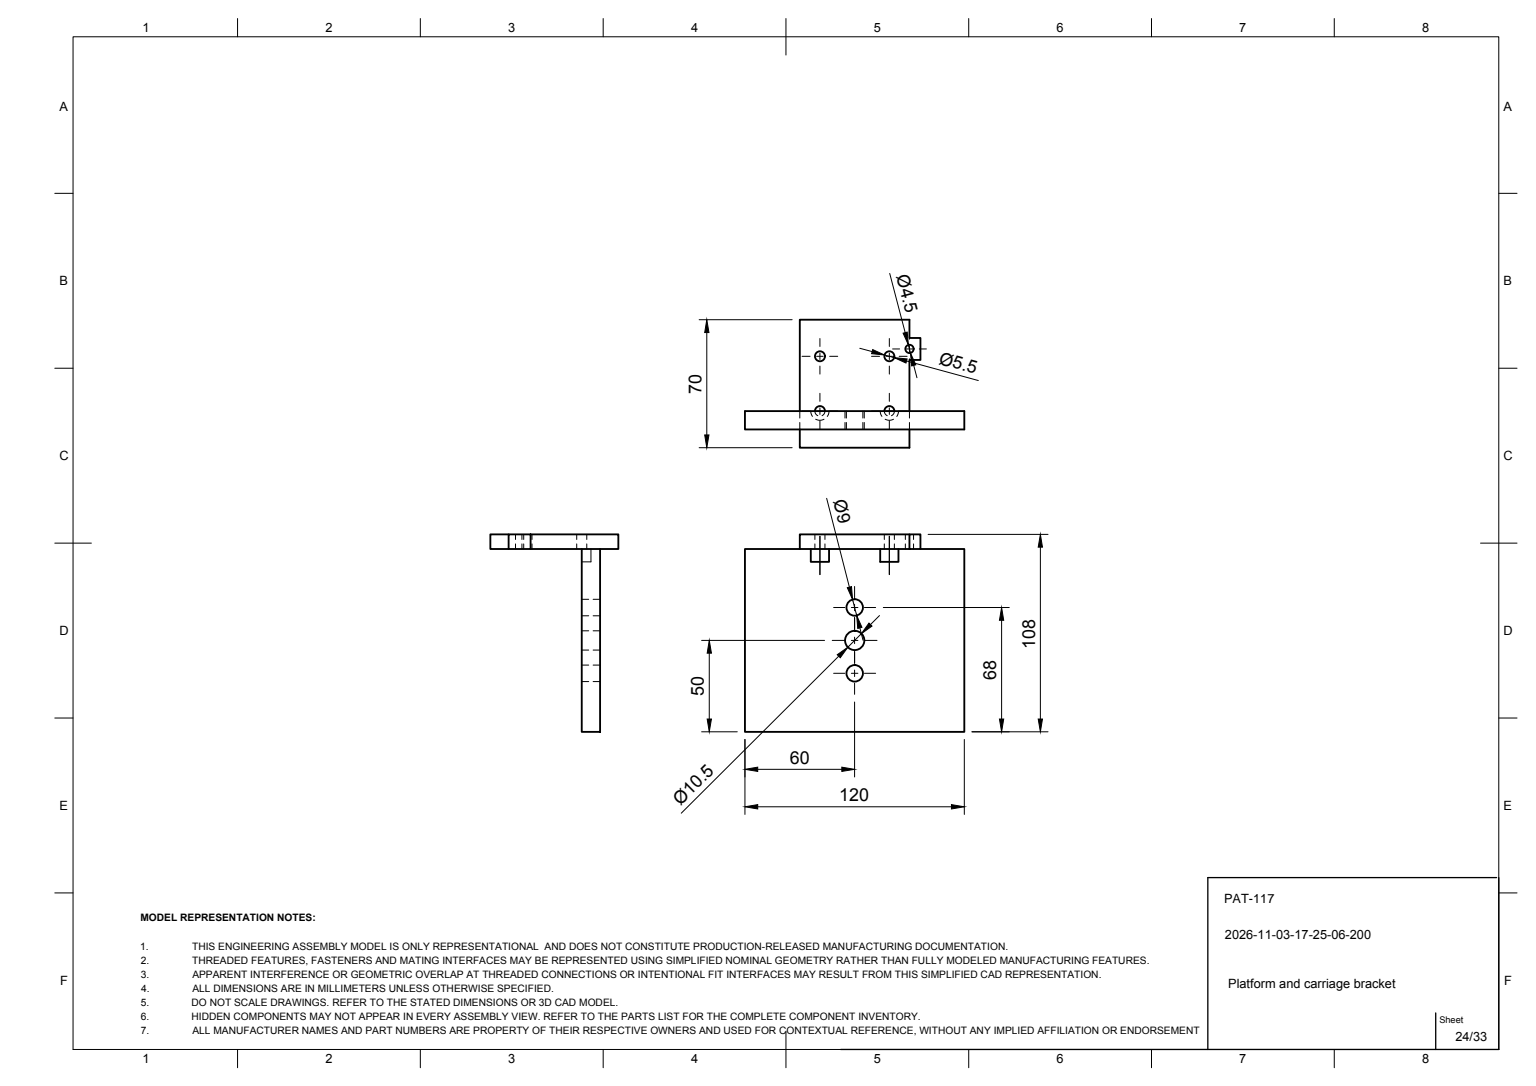
ISO-10303-21;
HEADER;
/* Generated by software containing ST-Developer
 * from STEP Tools, Inc. (www.steptools.com) 
 */

FILE_DESCRIPTION(
/* description */ ('Counterbalanced vertical column'),
/* implementation_level */ '2;1');

FILE_NAME(
/* name */ 'Platform and carriage bracket.step',
/* time_stamp */ '2026-10-29T16:47:22-07:00',
/* author */ (''),
/* organization */ (''),
/* preprocessor_version */ 'ST-DEVELOPER v20.2',
/* originating_system */ 'Autodesk Translation Framework v15.17.0.0',
/* authorisation */ '');

FILE_SCHEMA (('AUTOMOTIVE_DESIGN { 1 0 10303 214 3 1 1 }'));
ENDSEC;

DATA;
#10=MECHANICAL_DESIGN_GEOMETRIC_PRESENTATION_REPRESENTATION('',(#373),#15040);
#303=SHAPE_REPRESENTATION_RELATIONSHIP('SRR','None',#15208,#338);
#338=ADVANCED_BREP_SHAPE_REPRESENTATION('',(#406),#15027);
#373=STYLED_ITEM('',(#15436),#406);
#406=MANIFOLD_SOLID_BREP('Body1',#7098);
#498=FACE_BOUND('',#1588,.T.);
#499=FACE_BOUND('',#1589,.T.);
#500=FACE_BOUND('',#1590,.T.);
#501=FACE_BOUND('',#1591,.T.);
#502=FACE_BOUND('',#1592,.T.);
#503=FACE_BOUND('',#1595,.T.);
#504=FACE_BOUND('',#1596,.T.);
#505=FACE_BOUND('',#1597,.T.);
#506=FACE_BOUND('',#1609,.T.);
#507=FACE_BOUND('',#1610,.T.);
#508=FACE_BOUND('',#1611,.T.);
#509=FACE_BOUND('',#1614,.T.);
#510=FACE_BOUND('',#1615,.T.);
#511=FACE_BOUND('',#1616,.T.);
#512=FACE_BOUND('',#1617,.T.);
#513=FACE_BOUND('',#1618,.T.);
#721=PLANE('',#7936);
#722=PLANE('',#7937);
#723=PLANE('',#7938);
#724=PLANE('',#7939);
#725=PLANE('',#7940);
#726=PLANE('',#7953);
#727=PLANE('',#7954);
#728=PLANE('',#7962);
#729=PLANE('',#7967);
#730=PLANE('',#7972);
#731=PLANE('',#7973);
#732=PLANE('',#7974);
#733=PLANE('',#7975);
#734=PLANE('',#7976);
#735=PLANE('',#7977);
#736=PLANE('',#7978);
#737=PLANE('',#7979);
#738=PLANE('',#7980);
#739=PLANE('',#7981);
#740=PLANE('',#7982);
#1089=FACE_OUTER_BOUND('',#1576,.T.);
#1090=FACE_OUTER_BOUND('',#1577,.T.);
#1091=FACE_OUTER_BOUND('',#1578,.T.);
#1092=FACE_OUTER_BOUND('',#1579,.T.);
#1093=FACE_OUTER_BOUND('',#1580,.T.);
#1094=FACE_OUTER_BOUND('',#1581,.T.);
#1095=FACE_OUTER_BOUND('',#1582,.T.);
#1096=FACE_OUTER_BOUND('',#1583,.T.);
#1097=FACE_OUTER_BOUND('',#1584,.T.);
#1098=FACE_OUTER_BOUND('',#1585,.T.);
#1099=FACE_OUTER_BOUND('',#1586,.T.);
#1100=FACE_OUTER_BOUND('',#1587,.T.);
#1101=FACE_OUTER_BOUND('',#1593,.T.);
#1102=FACE_OUTER_BOUND('',#1594,.T.);
#1103=FACE_OUTER_BOUND('',#1598,.T.);
#1104=FACE_OUTER_BOUND('',#1599,.T.);
#1105=FACE_OUTER_BOUND('',#1600,.T.);
#1106=FACE_OUTER_BOUND('',#1601,.T.);
#1107=FACE_OUTER_BOUND('',#1602,.T.);
#1108=FACE_OUTER_BOUND('',#1603,.T.);
#1109=FACE_OUTER_BOUND('',#1604,.T.);
#1110=FACE_OUTER_BOUND('',#1605,.T.);
#1111=FACE_OUTER_BOUND('',#1606,.T.);
#1112=FACE_OUTER_BOUND('',#1607,.T.);
#1113=FACE_OUTER_BOUND('',#1608,.T.);
#1114=FACE_OUTER_BOUND('',#1612,.T.);
#1115=FACE_OUTER_BOUND('',#1613,.T.);
#1116=FACE_OUTER_BOUND('',#1619,.T.);
#1117=FACE_OUTER_BOUND('',#1620,.T.);
#1118=FACE_OUTER_BOUND('',#1621,.T.);
#1576=EDGE_LOOP('',(#5930,#5931,#5932,#5933));
#1577=EDGE_LOOP('',(#5934,#5935,#5936,#5937));
#1578=EDGE_LOOP('',(#5938,#5939,#5940,#5941));
#1579=EDGE_LOOP('',(#5942,#5943,#5944,#5945));
#1580=EDGE_LOOP('',(#5946,#5947,#5948,#5949));
#1581=EDGE_LOOP('',(#5950,#5951,#5952,#5953,#5954,#5955));
#1582=EDGE_LOOP('',(#5956,#5957,#5958,#5959));
#1583=EDGE_LOOP('',(#5960,#5961,#5962,#5963));
#1584=EDGE_LOOP('',(#5964,#5965,#5966,#5967));
#1585=EDGE_LOOP('',(#5968,#5969,#5970,#5971));
#1586=EDGE_LOOP('',(#5972,#5973));
#1587=EDGE_LOOP('',(#5974,#5975,#5976,#5977,#5978,#5979,#5980,#5981,#5982,
#5983,#5984,#5985));
#1588=EDGE_LOOP('',(#5986));
#1589=EDGE_LOOP('',(#5987));
#1590=EDGE_LOOP('',(#5988));
#1591=EDGE_LOOP('',(#5989));
#1592=EDGE_LOOP('',(#5990));
#1593=EDGE_LOOP('',(#5991,#5992,#5993,#5994));
#1594=EDGE_LOOP('',(#5995,#5996,#5997,#5998,#5999,#6000,#6001,#6002,#6003,
#6004,#6005,#6006,#6007,#6008));
#1595=EDGE_LOOP('',(#6009));
#1596=EDGE_LOOP('',(#6010));
#1597=EDGE_LOOP('',(#6011));
#1598=EDGE_LOOP('',(#6012,#6013,#6014,#6015));
#1599=EDGE_LOOP('',(#6016,#6017,#6018,#6019));
#1600=EDGE_LOOP('',(#6020,#6021));
#1601=EDGE_LOOP('',(#6022,#6023,#6024,#6025));
#1602=EDGE_LOOP('',(#6026,#6027,#6028,#6029));
#1603=EDGE_LOOP('',(#6030,#6031,#6032,#6033));
#1604=EDGE_LOOP('',(#6034,#6035,#6036,#6037));
#1605=EDGE_LOOP('',(#6038,#6039,#6040,#6041));
#1606=EDGE_LOOP('',(#6042,#6043,#6044,#6045));
#1607=EDGE_LOOP('',(#6046,#6047,#6048,#6049));
#1608=EDGE_LOOP('',(#6050,#6051,#6052,#6053,#6054,#6055));
#1609=EDGE_LOOP('',(#6056));
#1610=EDGE_LOOP('',(#6057));
#1611=EDGE_LOOP('',(#6058));
#1612=EDGE_LOOP('',(#6059,#6060,#6061,#6062));
#1613=EDGE_LOOP('',(#6063,#6064,#6065,#6066,#6067,#6068,#6069,#6070));
#1614=EDGE_LOOP('',(#6071));
#1615=EDGE_LOOP('',(#6072));
#1616=EDGE_LOOP('',(#6073));
#1617=EDGE_LOOP('',(#6074));
#1618=EDGE_LOOP('',(#6075));
#1619=EDGE_LOOP('',(#6076,#6077,#6078,#6079,#6080,#6081));
#1620=EDGE_LOOP('',(#6082,#6083,#6084,#6085));
#1621=EDGE_LOOP('',(#6086,#6087,#6088,#6089));
#2175=LINE('',#14219,#2846);
#2176=LINE('',#14224,#2847);
#2177=LINE('',#14226,#2848);
#2178=LINE('',#14228,#2849);
#2179=LINE('',#14229,#2850);
#2180=LINE('',#14232,#2851);
#2181=LINE('',#14234,#2852);
#2182=LINE('',#14235,#2853);
#2183=LINE('',#14239,#2854);
#2184=LINE('',#14240,#2855);
#2185=LINE('',#14241,#2856);
#2186=LINE('',#14244,#2857);
#2187=LINE('',#14246,#2858);
#2188=LINE('',#14247,#2859);
#2189=LINE('',#14250,#2860);
#2190=LINE('',#14252,#2861);
#2191=LINE('',#14254,#2862);
#2192=LINE('',#14256,#2863);
#2193=LINE('',#14257,#2864);
#2194=LINE('',#14262,#2865);
#2195=LINE('',#14268,#2866);
#2196=LINE('',#14274,#2867);
#2197=LINE('',#14279,#2868);
#2198=LINE('',#14283,#2869);
#2199=LINE('',#14286,#2870);
#2200=LINE('',#14289,#2871);
#2201=LINE('',#14291,#2872);
#2202=LINE('',#14293,#2873);
#2203=LINE('',#14296,#2874);
#2204=LINE('',#14297,#2875);
#2205=LINE('',#14308,#2876);
#2206=LINE('',#14312,#2877);
#2207=LINE('',#14314,#2878);
#2208=LINE('',#14315,#2879);
#2209=LINE('',#14317,#2880);
#2210=LINE('',#14319,#2881);
#2211=LINE('',#14321,#2882);
#2212=LINE('',#14323,#2883);
#2213=LINE('',#14324,#2884);
#2214=LINE('',#14327,#2885);
#2215=LINE('',#14334,#2886);
#2216=LINE('',#14338,#2887);
#2217=LINE('',#14342,#2888);
#2218=LINE('',#14344,#2889);
#2219=LINE('',#14345,#2890);
#2220=LINE('',#14348,#2891);
#2221=LINE('',#14349,#2892);
#2222=LINE('',#14352,#2893);
#2223=LINE('',#14353,#2894);
#2224=LINE('',#14356,#2895);
#2225=LINE('',#14357,#2896);
#2226=LINE('',#14359,#2897);
#2227=LINE('',#14361,#2898);
#2228=LINE('',#14364,#2899);
#2229=LINE('',#14365,#2900);
#2230=LINE('',#14368,#2901);
#2231=LINE('',#14370,#2902);
#2232=LINE('',#14371,#2903);
#2233=LINE('',#14373,#2904);
#2234=LINE('',#14374,#2905);
#2846=VECTOR('',#9519,0.225000000000001);
#2847=VECTOR('',#9524,1.);
#2848=VECTOR('',#9525,1.);
#2849=VECTOR('',#9526,1.);
#2850=VECTOR('',#9527,1.);
#2851=VECTOR('',#9530,1.);
#2852=VECTOR('',#9531,1.);
#2853=VECTOR('',#9532,1.);
#2854=VECTOR('',#9535,1.);
#2855=VECTOR('',#9536,1.);
#2856=VECTOR('',#9537,1.);
#2857=VECTOR('',#9540,1.);
#2858=VECTOR('',#9541,1.);
#2859=VECTOR('',#9542,1.);
#2860=VECTOR('',#9545,1.);
#2861=VECTOR('',#9546,1.);
#2862=VECTOR('',#9547,1.);
#2863=VECTOR('',#9548,1.);
#2864=VECTOR('',#9549,1.);
#2865=VECTOR('',#9554,0.525);
#2866=VECTOR('',#9561,0.45);
#2867=VECTOR('',#9568,0.449999999999999);
#2868=VECTOR('',#9573,1.);
#2869=VECTOR('',#9576,1.);
#2870=VECTOR('',#9581,1.);
#2871=VECTOR('',#9584,1.);
#2872=VECTOR('',#9585,1.);
#2873=VECTOR('',#9586,1.);
#2874=VECTOR('',#9589,1.);
#2875=VECTOR('',#9590,1.);
#2876=VECTOR('',#9601,0.274999999999999);
#2877=VECTOR('',#9606,1.);
#2878=VECTOR('',#9607,1.);
#2879=VECTOR('',#9608,1.);
#2880=VECTOR('',#9609,1.);
#2881=VECTOR('',#9610,1.);
#2882=VECTOR('',#9611,1.);
#2883=VECTOR('',#9612,1.);
#2884=VECTOR('',#9613,1.);
#2885=VECTOR('',#9616,0.274999999999999);
#2886=VECTOR('',#9627,0.274999999999999);
#2887=VECTOR('',#9632,0.274999999999999);
#2888=VECTOR('',#9637,1.);
#2889=VECTOR('',#9638,1.);
#2890=VECTOR('',#9639,1.);
#2891=VECTOR('',#9642,1.);
#2892=VECTOR('',#9643,1.);
#2893=VECTOR('',#9646,1.);
#2894=VECTOR('',#9647,1.);
#2895=VECTOR('',#9650,1.);
#2896=VECTOR('',#9651,1.);
#2897=VECTOR('',#9654,1.);
#2898=VECTOR('',#9657,1.);
#2899=VECTOR('',#9660,1.);
#2900=VECTOR('',#9661,1.);
#2901=VECTOR('',#9664,1.);
#2902=VECTOR('',#9665,1.);
#2903=VECTOR('',#9666,1.);
#2904=VECTOR('',#9669,1.);
#2905=VECTOR('',#9670,1.);
#3231=CIRCLE('',#7934,0.225000000000001);
#3232=CIRCLE('',#7935,0.225000000000001);
#3233=CIRCLE('',#7942,0.525);
#3234=CIRCLE('',#7943,0.525);
#3235=CIRCLE('',#7945,0.45);
#3236=CIRCLE('',#7946,0.45);
#3237=CIRCLE('',#7948,0.449999999999999);
#3238=CIRCLE('',#7949,0.449999999999999);
#3239=CIRCLE('',#7951,0.5);
#3240=CIRCLE('',#7952,0.5);
#3241=CIRCLE('',#7955,0.5);
#3242=CIRCLE('',#7956,0.274999999999999);
#3243=CIRCLE('',#7957,0.274999999999999);
#3244=CIRCLE('',#7958,0.274999999999999);
#3245=CIRCLE('',#7959,0.274999999999999);
#3246=CIRCLE('',#7961,0.274999999999999);
#3247=CIRCLE('',#7964,0.274999999999999);
#3248=CIRCLE('',#7966,0.5);
#3249=CIRCLE('',#7969,0.274999999999999);
#3250=CIRCLE('',#7971,0.274999999999999);
#3684=VERTEX_POINT('',#14216);
#3685=VERTEX_POINT('',#14218);
#3686=VERTEX_POINT('',#14222);
#3687=VERTEX_POINT('',#14223);
#3688=VERTEX_POINT('',#14225);
#3689=VERTEX_POINT('',#14227);
#3690=VERTEX_POINT('',#14231);
#3691=VERTEX_POINT('',#14233);
#3692=VERTEX_POINT('',#14237);
#3693=VERTEX_POINT('',#14238);
#3694=VERTEX_POINT('',#14243);
#3695=VERTEX_POINT('',#14245);
#3696=VERTEX_POINT('',#14249);
#3697=VERTEX_POINT('',#14251);
#3698=VERTEX_POINT('',#14253);
#3699=VERTEX_POINT('',#14255);
#3700=VERTEX_POINT('',#14259);
#3701=VERTEX_POINT('',#14261);
#3702=VERTEX_POINT('',#14265);
#3703=VERTEX_POINT('',#14267);
#3704=VERTEX_POINT('',#14271);
#3705=VERTEX_POINT('',#14273);
#3706=VERTEX_POINT('',#14277);
#3707=VERTEX_POINT('',#14278);
#3708=VERTEX_POINT('',#14280);
#3709=VERTEX_POINT('',#14282);
#3710=VERTEX_POINT('',#14288);
#3711=VERTEX_POINT('',#14290);
#3712=VERTEX_POINT('',#14292);
#3713=VERTEX_POINT('',#14294);
#3714=VERTEX_POINT('',#14298);
#3715=VERTEX_POINT('',#14300);
#3716=VERTEX_POINT('',#14302);
#3717=VERTEX_POINT('',#14304);
#3718=VERTEX_POINT('',#14307);
#3719=VERTEX_POINT('',#14311);
#3720=VERTEX_POINT('',#14313);
#3721=VERTEX_POINT('',#14316);
#3722=VERTEX_POINT('',#14318);
#3723=VERTEX_POINT('',#14320);
#3724=VERTEX_POINT('',#14322);
#3725=VERTEX_POINT('',#14326);
#3726=VERTEX_POINT('',#14333);
#3727=VERTEX_POINT('',#14337);
#3728=VERTEX_POINT('',#14341);
#3729=VERTEX_POINT('',#14343);
#3730=VERTEX_POINT('',#14347);
#3731=VERTEX_POINT('',#14351);
#3732=VERTEX_POINT('',#14355);
#3733=VERTEX_POINT('',#14363);
#3734=VERTEX_POINT('',#14367);
#3735=VERTEX_POINT('',#14369);
#4466=EDGE_CURVE('',#3684,#3684,#3231,.T.);
#4467=EDGE_CURVE('',#3684,#3685,#2175,.T.);
#4468=EDGE_CURVE('',#3685,#3685,#3232,.T.);
#4469=EDGE_CURVE('',#3686,#3687,#2176,.T.);
#4470=EDGE_CURVE('',#3688,#3686,#2177,.T.);
#4471=EDGE_CURVE('',#3689,#3688,#2178,.T.);
#4472=EDGE_CURVE('',#3687,#3689,#2179,.T.);
#4473=EDGE_CURVE('',#3688,#3690,#2180,.T.);
#4474=EDGE_CURVE('',#3691,#3690,#2181,.T.);
#4475=EDGE_CURVE('',#3689,#3691,#2182,.T.);
#4476=EDGE_CURVE('',#3692,#3693,#2183,.T.);
#4477=EDGE_CURVE('',#3692,#3691,#2184,.T.);
#4478=EDGE_CURVE('',#3690,#3693,#2185,.T.);
#4479=EDGE_CURVE('',#3694,#3687,#2186,.T.);
#4480=EDGE_CURVE('',#3694,#3695,#2187,.T.);
#4481=EDGE_CURVE('',#3695,#3686,#2188,.T.);
#4482=EDGE_CURVE('',#3693,#3696,#2189,.T.);
#4483=EDGE_CURVE('',#3696,#3697,#2190,.T.);
#4484=EDGE_CURVE('',#3697,#3698,#2191,.T.);
#4485=EDGE_CURVE('',#3699,#3698,#2192,.T.);
#4486=EDGE_CURVE('',#3692,#3699,#2193,.T.);
#4487=EDGE_CURVE('',#3700,#3700,#3233,.T.);
#4488=EDGE_CURVE('',#3700,#3701,#2194,.T.);
#4489=EDGE_CURVE('',#3701,#3701,#3234,.T.);
#4490=EDGE_CURVE('',#3702,#3702,#3235,.T.);
#4491=EDGE_CURVE('',#3702,#3703,#2195,.T.);
#4492=EDGE_CURVE('',#3703,#3703,#3236,.T.);
#4493=EDGE_CURVE('',#3704,#3704,#3237,.T.);
#4494=EDGE_CURVE('',#3704,#3705,#2196,.T.);
#4495=EDGE_CURVE('',#3705,#3705,#3238,.T.);
#4496=EDGE_CURVE('',#3706,#3707,#2197,.T.);
#4497=EDGE_CURVE('',#3708,#3706,#3239,.T.);
#4498=EDGE_CURVE('',#3709,#3708,#2198,.T.);
#4499=EDGE_CURVE('',#3709,#3707,#3240,.T.);
#4500=EDGE_CURVE('',#3708,#3706,#2199,.T.);
#4501=EDGE_CURVE('',#3695,#3710,#2200,.T.);
#4502=EDGE_CURVE('',#3710,#3711,#2201,.T.);
#4503=EDGE_CURVE('',#3711,#3712,#2202,.T.);
#4504=EDGE_CURVE('',#3713,#3712,#3241,.T.);
#4505=EDGE_CURVE('',#3713,#3707,#2203,.T.);
#4506=EDGE_CURVE('',#3709,#3696,#2204,.T.);
#4507=EDGE_CURVE('',#3714,#3714,#3242,.T.);
#4508=EDGE_CURVE('',#3715,#3715,#3243,.T.);
#4509=EDGE_CURVE('',#3716,#3716,#3244,.T.);
#4510=EDGE_CURVE('',#3717,#3717,#3245,.T.);
#4511=EDGE_CURVE('',#3714,#3718,#2205,.T.);
#4512=EDGE_CURVE('',#3718,#3718,#3246,.T.);
#4513=EDGE_CURVE('',#3713,#3719,#2206,.T.);
#4514=EDGE_CURVE('',#3719,#3720,#2207,.T.);
#4515=EDGE_CURVE('',#3720,#3712,#2208,.T.);
#4516=EDGE_CURVE('',#3721,#3711,#2209,.T.);
#4517=EDGE_CURVE('',#3722,#3721,#2210,.T.);
#4518=EDGE_CURVE('',#3723,#3722,#2211,.T.);
#4519=EDGE_CURVE('',#3724,#3723,#2212,.T.);
#4520=EDGE_CURVE('',#3696,#3724,#2213,.T.);
#4521=EDGE_CURVE('',#3717,#3725,#2214,.T.);
#4522=EDGE_CURVE('',#3725,#3725,#3247,.T.);
#4523=EDGE_CURVE('',#3719,#3720,#3248,.T.);
#4524=EDGE_CURVE('',#3716,#3726,#2215,.T.);
#4525=EDGE_CURVE('',#3726,#3726,#3249,.T.);
#4526=EDGE_CURVE('',#3715,#3727,#2216,.T.);
#4527=EDGE_CURVE('',#3727,#3727,#3250,.T.);
#4528=EDGE_CURVE('',#3711,#3728,#2217,.T.);
#4529=EDGE_CURVE('',#3729,#3728,#2218,.T.);
#4530=EDGE_CURVE('',#3721,#3729,#2219,.T.);
#4531=EDGE_CURVE('',#3724,#3730,#2220,.T.);
#4532=EDGE_CURVE('',#3697,#3730,#2221,.T.);
#4533=EDGE_CURVE('',#3723,#3731,#2222,.T.);
#4534=EDGE_CURVE('',#3730,#3731,#2223,.T.);
#4535=EDGE_CURVE('',#3732,#3729,#2224,.T.);
#4536=EDGE_CURVE('',#3722,#3732,#2225,.T.);
#4537=EDGE_CURVE('',#3731,#3732,#2226,.T.);
#4538=EDGE_CURVE('',#3697,#3728,#2227,.T.);
#4539=EDGE_CURVE('',#3728,#3733,#2228,.T.);
#4540=EDGE_CURVE('',#3698,#3733,#2229,.T.);
#4541=EDGE_CURVE('',#3734,#3699,#2230,.T.);
#4542=EDGE_CURVE('',#3735,#3734,#2231,.T.);
#4543=EDGE_CURVE('',#3735,#3694,#2232,.T.);
#4544=EDGE_CURVE('',#3710,#3735,#2233,.T.);
#4545=EDGE_CURVE('',#3733,#3734,#2234,.T.);
#5930=ORIENTED_EDGE('',*,*,#4466,.F.);
#5931=ORIENTED_EDGE('',*,*,#4467,.T.);
#5932=ORIENTED_EDGE('',*,*,#4468,.F.);
#5933=ORIENTED_EDGE('',*,*,#4467,.F.);
#5934=ORIENTED_EDGE('',*,*,#4469,.F.);
#5935=ORIENTED_EDGE('',*,*,#4470,.F.);
#5936=ORIENTED_EDGE('',*,*,#4471,.F.);
#5937=ORIENTED_EDGE('',*,*,#4472,.F.);
#5938=ORIENTED_EDGE('',*,*,#4471,.T.);
#5939=ORIENTED_EDGE('',*,*,#4473,.T.);
#5940=ORIENTED_EDGE('',*,*,#4474,.F.);
#5941=ORIENTED_EDGE('',*,*,#4475,.F.);
#5942=ORIENTED_EDGE('',*,*,#4476,.F.);
#5943=ORIENTED_EDGE('',*,*,#4477,.T.);
#5944=ORIENTED_EDGE('',*,*,#4474,.T.);
#5945=ORIENTED_EDGE('',*,*,#4478,.T.);
#5946=ORIENTED_EDGE('',*,*,#4469,.T.);
#5947=ORIENTED_EDGE('',*,*,#4479,.F.);
#5948=ORIENTED_EDGE('',*,*,#4480,.T.);
#5949=ORIENTED_EDGE('',*,*,#4481,.T.);
#5950=ORIENTED_EDGE('',*,*,#4476,.T.);
#5951=ORIENTED_EDGE('',*,*,#4482,.T.);
#5952=ORIENTED_EDGE('',*,*,#4483,.T.);
#5953=ORIENTED_EDGE('',*,*,#4484,.T.);
#5954=ORIENTED_EDGE('',*,*,#4485,.F.);
#5955=ORIENTED_EDGE('',*,*,#4486,.F.);
#5956=ORIENTED_EDGE('',*,*,#4487,.F.);
#5957=ORIENTED_EDGE('',*,*,#4488,.T.);
#5958=ORIENTED_EDGE('',*,*,#4489,.F.);
#5959=ORIENTED_EDGE('',*,*,#4488,.F.);
#5960=ORIENTED_EDGE('',*,*,#4490,.F.);
#5961=ORIENTED_EDGE('',*,*,#4491,.T.);
#5962=ORIENTED_EDGE('',*,*,#4492,.F.);
#5963=ORIENTED_EDGE('',*,*,#4491,.F.);
#5964=ORIENTED_EDGE('',*,*,#4493,.F.);
#5965=ORIENTED_EDGE('',*,*,#4494,.T.);
#5966=ORIENTED_EDGE('',*,*,#4495,.F.);
#5967=ORIENTED_EDGE('',*,*,#4494,.F.);
#5968=ORIENTED_EDGE('',*,*,#4496,.F.);
#5969=ORIENTED_EDGE('',*,*,#4497,.F.);
#5970=ORIENTED_EDGE('',*,*,#4498,.F.);
#5971=ORIENTED_EDGE('',*,*,#4499,.T.);
#5972=ORIENTED_EDGE('',*,*,#4500,.F.);
#5973=ORIENTED_EDGE('',*,*,#4497,.T.);
#5974=ORIENTED_EDGE('',*,*,#4481,.F.);
#5975=ORIENTED_EDGE('',*,*,#4501,.T.);
#5976=ORIENTED_EDGE('',*,*,#4502,.T.);
#5977=ORIENTED_EDGE('',*,*,#4503,.T.);
#5978=ORIENTED_EDGE('',*,*,#4504,.F.);
#5979=ORIENTED_EDGE('',*,*,#4505,.T.);
#5980=ORIENTED_EDGE('',*,*,#4499,.F.);
#5981=ORIENTED_EDGE('',*,*,#4506,.T.);
#5982=ORIENTED_EDGE('',*,*,#4482,.F.);
#5983=ORIENTED_EDGE('',*,*,#4478,.F.);
#5984=ORIENTED_EDGE('',*,*,#4473,.F.);
#5985=ORIENTED_EDGE('',*,*,#4470,.T.);
#5986=ORIENTED_EDGE('',*,*,#4466,.T.);
#5987=ORIENTED_EDGE('',*,*,#4507,.T.);
#5988=ORIENTED_EDGE('',*,*,#4508,.T.);
#5989=ORIENTED_EDGE('',*,*,#4509,.F.);
#5990=ORIENTED_EDGE('',*,*,#4510,.T.);
#5991=ORIENTED_EDGE('',*,*,#4507,.F.);
#5992=ORIENTED_EDGE('',*,*,#4511,.T.);
#5993=ORIENTED_EDGE('',*,*,#4512,.F.);
#5994=ORIENTED_EDGE('',*,*,#4511,.F.);
#5995=ORIENTED_EDGE('',*,*,#4496,.T.);
#5996=ORIENTED_EDGE('',*,*,#4505,.F.);
#5997=ORIENTED_EDGE('',*,*,#4513,.T.);
#5998=ORIENTED_EDGE('',*,*,#4514,.T.);
#5999=ORIENTED_EDGE('',*,*,#4515,.T.);
#6000=ORIENTED_EDGE('',*,*,#4503,.F.);
#6001=ORIENTED_EDGE('',*,*,#4516,.F.);
#6002=ORIENTED_EDGE('',*,*,#4517,.F.);
#6003=ORIENTED_EDGE('',*,*,#4518,.F.);
#6004=ORIENTED_EDGE('',*,*,#4519,.F.);
#6005=ORIENTED_EDGE('',*,*,#4520,.F.);
#6006=ORIENTED_EDGE('',*,*,#4506,.F.);
#6007=ORIENTED_EDGE('',*,*,#4498,.T.);
#6008=ORIENTED_EDGE('',*,*,#4500,.T.);
#6009=ORIENTED_EDGE('',*,*,#4487,.T.);
#6010=ORIENTED_EDGE('',*,*,#4490,.T.);
#6011=ORIENTED_EDGE('',*,*,#4493,.T.);
#6012=ORIENTED_EDGE('',*,*,#4510,.F.);
#6013=ORIENTED_EDGE('',*,*,#4521,.T.);
#6014=ORIENTED_EDGE('',*,*,#4522,.F.);
#6015=ORIENTED_EDGE('',*,*,#4521,.F.);
#6016=ORIENTED_EDGE('',*,*,#4515,.F.);
#6017=ORIENTED_EDGE('',*,*,#4523,.F.);
#6018=ORIENTED_EDGE('',*,*,#4513,.F.);
#6019=ORIENTED_EDGE('',*,*,#4504,.T.);
#6020=ORIENTED_EDGE('',*,*,#4514,.F.);
#6021=ORIENTED_EDGE('',*,*,#4523,.T.);
#6022=ORIENTED_EDGE('',*,*,#4509,.T.);
#6023=ORIENTED_EDGE('',*,*,#4524,.T.);
#6024=ORIENTED_EDGE('',*,*,#4525,.F.);
#6025=ORIENTED_EDGE('',*,*,#4524,.F.);
#6026=ORIENTED_EDGE('',*,*,#4508,.F.);
#6027=ORIENTED_EDGE('',*,*,#4526,.T.);
#6028=ORIENTED_EDGE('',*,*,#4527,.F.);
#6029=ORIENTED_EDGE('',*,*,#4526,.F.);
#6030=ORIENTED_EDGE('',*,*,#4528,.T.);
#6031=ORIENTED_EDGE('',*,*,#4529,.F.);
#6032=ORIENTED_EDGE('',*,*,#4530,.F.);
#6033=ORIENTED_EDGE('',*,*,#4516,.T.);
#6034=ORIENTED_EDGE('',*,*,#4483,.F.);
#6035=ORIENTED_EDGE('',*,*,#4520,.T.);
#6036=ORIENTED_EDGE('',*,*,#4531,.T.);
#6037=ORIENTED_EDGE('',*,*,#4532,.F.);
#6038=ORIENTED_EDGE('',*,*,#4519,.T.);
#6039=ORIENTED_EDGE('',*,*,#4533,.T.);
#6040=ORIENTED_EDGE('',*,*,#4534,.F.);
#6041=ORIENTED_EDGE('',*,*,#4531,.F.);
#6042=ORIENTED_EDGE('',*,*,#4517,.T.);
#6043=ORIENTED_EDGE('',*,*,#4530,.T.);
#6044=ORIENTED_EDGE('',*,*,#4535,.F.);
#6045=ORIENTED_EDGE('',*,*,#4536,.F.);
#6046=ORIENTED_EDGE('',*,*,#4518,.T.);
#6047=ORIENTED_EDGE('',*,*,#4536,.T.);
#6048=ORIENTED_EDGE('',*,*,#4537,.F.);
#6049=ORIENTED_EDGE('',*,*,#4533,.F.);
#6050=ORIENTED_EDGE('',*,*,#4537,.T.);
#6051=ORIENTED_EDGE('',*,*,#4535,.T.);
#6052=ORIENTED_EDGE('',*,*,#4529,.T.);
#6053=ORIENTED_EDGE('',*,*,#4538,.F.);
#6054=ORIENTED_EDGE('',*,*,#4532,.T.);
#6055=ORIENTED_EDGE('',*,*,#4534,.T.);
#6056=ORIENTED_EDGE('',*,*,#4489,.T.);
#6057=ORIENTED_EDGE('',*,*,#4492,.T.);
#6058=ORIENTED_EDGE('',*,*,#4495,.T.);
#6059=ORIENTED_EDGE('',*,*,#4538,.T.);
#6060=ORIENTED_EDGE('',*,*,#4539,.T.);
#6061=ORIENTED_EDGE('',*,*,#4540,.F.);
#6062=ORIENTED_EDGE('',*,*,#4484,.F.);
#6063=ORIENTED_EDGE('',*,*,#4486,.T.);
#6064=ORIENTED_EDGE('',*,*,#4541,.F.);
#6065=ORIENTED_EDGE('',*,*,#4542,.F.);
#6066=ORIENTED_EDGE('',*,*,#4543,.T.);
#6067=ORIENTED_EDGE('',*,*,#4479,.T.);
#6068=ORIENTED_EDGE('',*,*,#4472,.T.);
#6069=ORIENTED_EDGE('',*,*,#4475,.T.);
#6070=ORIENTED_EDGE('',*,*,#4477,.F.);
#6071=ORIENTED_EDGE('',*,*,#4468,.T.);
#6072=ORIENTED_EDGE('',*,*,#4512,.T.);
#6073=ORIENTED_EDGE('',*,*,#4522,.T.);
#6074=ORIENTED_EDGE('',*,*,#4525,.T.);
#6075=ORIENTED_EDGE('',*,*,#4527,.T.);
#6076=ORIENTED_EDGE('',*,*,#4544,.T.);
#6077=ORIENTED_EDGE('',*,*,#4542,.T.);
#6078=ORIENTED_EDGE('',*,*,#4545,.F.);
#6079=ORIENTED_EDGE('',*,*,#4539,.F.);
#6080=ORIENTED_EDGE('',*,*,#4528,.F.);
#6081=ORIENTED_EDGE('',*,*,#4502,.F.);
#6082=ORIENTED_EDGE('',*,*,#4540,.T.);
#6083=ORIENTED_EDGE('',*,*,#4545,.T.);
#6084=ORIENTED_EDGE('',*,*,#4541,.T.);
#6085=ORIENTED_EDGE('',*,*,#4485,.T.);
#6086=ORIENTED_EDGE('',*,*,#4501,.F.);
#6087=ORIENTED_EDGE('',*,*,#4480,.F.);
#6088=ORIENTED_EDGE('',*,*,#4543,.F.);
#6089=ORIENTED_EDGE('',*,*,#4544,.F.);
#6638=CYLINDRICAL_SURFACE('',#7933,0.225000000000001);
#6639=CYLINDRICAL_SURFACE('',#7941,0.525);
#6640=CYLINDRICAL_SURFACE('',#7944,0.45);
#6641=CYLINDRICAL_SURFACE('',#7947,0.449999999999999);
#6642=CYLINDRICAL_SURFACE('',#7950,0.5);
#6643=CYLINDRICAL_SURFACE('',#7960,0.274999999999999);
#6644=CYLINDRICAL_SURFACE('',#7963,0.274999999999999);
#6645=CYLINDRICAL_SURFACE('',#7965,0.5);
#6646=CYLINDRICAL_SURFACE('',#7968,0.274999999999999);
#6647=CYLINDRICAL_SURFACE('',#7970,0.274999999999999);
#6931=ADVANCED_FACE('',(#1089),#6638,.F.);
#6932=ADVANCED_FACE('',(#1090),#721,.F.);
#6933=ADVANCED_FACE('',(#1091),#722,.T.);
#6934=ADVANCED_FACE('',(#1092),#723,.T.);
#6935=ADVANCED_FACE('',(#1093),#724,.T.);
#6936=ADVANCED_FACE('',(#1094),#725,.T.);
#6937=ADVANCED_FACE('',(#1095),#6639,.F.);
#6938=ADVANCED_FACE('',(#1096),#6640,.F.);
#6939=ADVANCED_FACE('',(#1097),#6641,.F.);
#6940=ADVANCED_FACE('',(#1098),#6642,.F.);
#6941=ADVANCED_FACE('',(#1099),#726,.T.);
#6942=ADVANCED_FACE('',(#1100,#498,#499,#500,#501,#502),#727,.T.);
#6943=ADVANCED_FACE('',(#1101),#6643,.F.);
#6944=ADVANCED_FACE('',(#1102,#503,#504,#505),#728,.F.);
#6945=ADVANCED_FACE('',(#1103),#6644,.F.);
#6946=ADVANCED_FACE('',(#1104),#6645,.F.);
#6947=ADVANCED_FACE('',(#1105),#729,.T.);
#6948=ADVANCED_FACE('',(#1106),#6646,.F.);
#6949=ADVANCED_FACE('',(#1107),#6647,.F.);
#6950=ADVANCED_FACE('',(#1108),#730,.T.);
#6951=ADVANCED_FACE('',(#1109),#731,.T.);
#6952=ADVANCED_FACE('',(#1110),#732,.T.);
#6953=ADVANCED_FACE('',(#1111),#733,.T.);
#6954=ADVANCED_FACE('',(#1112),#734,.T.);
#6955=ADVANCED_FACE('',(#1113,#506,#507,#508),#735,.T.);
#6956=ADVANCED_FACE('',(#1114),#736,.T.);
#6957=ADVANCED_FACE('',(#1115,#509,#510,#511,#512,#513),#737,.T.);
#6958=ADVANCED_FACE('',(#1116),#738,.T.);
#6959=ADVANCED_FACE('',(#1117),#739,.T.);
#6960=ADVANCED_FACE('',(#1118),#740,.F.);
#7098=CLOSED_SHELL('',(#6931,#6932,#6933,#6934,#6935,#6936,#6937,#6938,
#6939,#6940,#6941,#6942,#6943,#6944,#6945,#6946,#6947,#6948,#6949,#6950,
#6951,#6952,#6953,#6954,#6955,#6956,#6957,#6958,#6959,#6960));
#7932=AXIS2_PLACEMENT_3D('',#14214,#9513,#9514);
#7933=AXIS2_PLACEMENT_3D('',#14215,#9515,#9516);
#7934=AXIS2_PLACEMENT_3D('',#14217,#9517,#9518);
#7935=AXIS2_PLACEMENT_3D('',#14220,#9520,#9521);
#7936=AXIS2_PLACEMENT_3D('',#14221,#9522,#9523);
#7937=AXIS2_PLACEMENT_3D('',#14230,#9528,#9529);
#7938=AXIS2_PLACEMENT_3D('',#14236,#9533,#9534);
#7939=AXIS2_PLACEMENT_3D('',#14242,#9538,#9539);
#7940=AXIS2_PLACEMENT_3D('',#14248,#9543,#9544);
#7941=AXIS2_PLACEMENT_3D('',#14258,#9550,#9551);
#7942=AXIS2_PLACEMENT_3D('',#14260,#9552,#9553);
#7943=AXIS2_PLACEMENT_3D('',#14263,#9555,#9556);
#7944=AXIS2_PLACEMENT_3D('',#14264,#9557,#9558);
#7945=AXIS2_PLACEMENT_3D('',#14266,#9559,#9560);
#7946=AXIS2_PLACEMENT_3D('',#14269,#9562,#9563);
#7947=AXIS2_PLACEMENT_3D('',#14270,#9564,#9565);
#7948=AXIS2_PLACEMENT_3D('',#14272,#9566,#9567);
#7949=AXIS2_PLACEMENT_3D('',#14275,#9569,#9570);
#7950=AXIS2_PLACEMENT_3D('',#14276,#9571,#9572);
#7951=AXIS2_PLACEMENT_3D('',#14281,#9574,#9575);
#7952=AXIS2_PLACEMENT_3D('',#14284,#9577,#9578);
#7953=AXIS2_PLACEMENT_3D('',#14285,#9579,#9580);
#7954=AXIS2_PLACEMENT_3D('',#14287,#9582,#9583);
#7955=AXIS2_PLACEMENT_3D('',#14295,#9587,#9588);
#7956=AXIS2_PLACEMENT_3D('',#14299,#9591,#9592);
#7957=AXIS2_PLACEMENT_3D('',#14301,#9593,#9594);
#7958=AXIS2_PLACEMENT_3D('',#14303,#9595,#9596);
#7959=AXIS2_PLACEMENT_3D('',#14305,#9597,#9598);
#7960=AXIS2_PLACEMENT_3D('',#14306,#9599,#9600);
#7961=AXIS2_PLACEMENT_3D('',#14309,#9602,#9603);
#7962=AXIS2_PLACEMENT_3D('',#14310,#9604,#9605);
#7963=AXIS2_PLACEMENT_3D('',#14325,#9614,#9615);
#7964=AXIS2_PLACEMENT_3D('',#14328,#9617,#9618);
#7965=AXIS2_PLACEMENT_3D('',#14329,#9619,#9620);
#7966=AXIS2_PLACEMENT_3D('',#14330,#9621,#9622);
#7967=AXIS2_PLACEMENT_3D('',#14331,#9623,#9624);
#7968=AXIS2_PLACEMENT_3D('',#14332,#9625,#9626);
#7969=AXIS2_PLACEMENT_3D('',#14335,#9628,#9629);
#7970=AXIS2_PLACEMENT_3D('',#14336,#9630,#9631);
#7971=AXIS2_PLACEMENT_3D('',#14339,#9633,#9634);
#7972=AXIS2_PLACEMENT_3D('',#14340,#9635,#9636);
#7973=AXIS2_PLACEMENT_3D('',#14346,#9640,#9641);
#7974=AXIS2_PLACEMENT_3D('',#14350,#9644,#9645);
#7975=AXIS2_PLACEMENT_3D('',#14354,#9648,#9649);
#7976=AXIS2_PLACEMENT_3D('',#14358,#9652,#9653);
#7977=AXIS2_PLACEMENT_3D('',#14360,#9655,#9656);
#7978=AXIS2_PLACEMENT_3D('',#14362,#9658,#9659);
#7979=AXIS2_PLACEMENT_3D('',#14366,#9662,#9663);
#7980=AXIS2_PLACEMENT_3D('',#14372,#9667,#9668);
#7981=AXIS2_PLACEMENT_3D('',#14375,#9671,#9672);
#7982=AXIS2_PLACEMENT_3D('',#14376,#9673,#9674);
#9513=DIRECTION('axis',(0.,0.,1.));
#9514=DIRECTION('refdir',(1.,0.,0.));
#9515=DIRECTION('center_axis',(1.,0.,0.));
#9516=DIRECTION('ref_axis',(0.,0.,-1.));
#9517=DIRECTION('center_axis',(1.,0.,0.));
#9518=DIRECTION('ref_axis',(0.,0.,-1.));
#9519=DIRECTION('',(1.,0.,0.));
#9520=DIRECTION('center_axis',(-1.,0.,0.));
#9521=DIRECTION('ref_axis',(0.,0.,-1.));
#9522=DIRECTION('center_axis',(0.,0.,1.));
#9523=DIRECTION('ref_axis',(1.,0.,0.));
#9524=DIRECTION('',(1.,0.,0.));
#9525=DIRECTION('',(0.,-1.,0.));
#9526=DIRECTION('',(-1.,0.,0.));
#9527=DIRECTION('',(0.,1.,0.));
#9528=DIRECTION('center_axis',(0.,1.,0.));
#9529=DIRECTION('ref_axis',(-1.,0.,0.));
#9530=DIRECTION('',(0.,0.,1.));
#9531=DIRECTION('',(-1.,0.,0.));
#9532=DIRECTION('',(0.,0.,1.));
#9533=DIRECTION('center_axis',(0.,0.,1.));
#9534=DIRECTION('ref_axis',(1.,0.,0.));
#9535=DIRECTION('',(-1.,0.,0.));
#9536=DIRECTION('',(0.,1.,0.));
#9537=DIRECTION('',(0.,-1.,0.));
#9538=DIRECTION('center_axis',(0.,1.,0.));
#9539=DIRECTION('ref_axis',(-1.,0.,0.));
#9540=DIRECTION('',(0.,0.,1.));
#9541=DIRECTION('',(-1.,0.,0.));
#9542=DIRECTION('',(0.,0.,1.));
#9543=DIRECTION('center_axis',(0.,1.,0.));
#9544=DIRECTION('ref_axis',(-1.,0.,0.));
#9545=DIRECTION('',(0.,0.,1.));
#9546=DIRECTION('',(0.,0.,1.));
#9547=DIRECTION('',(0.,0.,1.));
#9548=DIRECTION('',(-1.,0.,0.));
#9549=DIRECTION('',(0.,0.,1.));
#9550=DIRECTION('center_axis',(0.,0.,1.));
#9551=DIRECTION('ref_axis',(1.,0.,0.));
#9552=DIRECTION('center_axis',(0.,0.,1.));
#9553=DIRECTION('ref_axis',(1.,0.,0.));
#9554=DIRECTION('',(0.,0.,1.));
#9555=DIRECTION('center_axis',(0.,0.,-1.));
#9556=DIRECTION('ref_axis',(1.,0.,0.));
#9557=DIRECTION('center_axis',(0.,0.,1.));
#9558=DIRECTION('ref_axis',(1.,0.,0.));
#9559=DIRECTION('center_axis',(0.,0.,1.));
#9560=DIRECTION('ref_axis',(1.,0.,0.));
#9561=DIRECTION('',(0.,0.,1.));
#9562=DIRECTION('center_axis',(0.,0.,-1.));
#9563=DIRECTION('ref_axis',(1.,0.,0.));
#9564=DIRECTION('center_axis',(0.,0.,1.));
#9565=DIRECTION('ref_axis',(1.,0.,0.));
#9566=DIRECTION('center_axis',(0.,0.,1.));
#9567=DIRECTION('ref_axis',(1.,0.,0.));
#9568=DIRECTION('',(0.,0.,1.));
#9569=DIRECTION('center_axis',(0.,0.,-1.));
#9570=DIRECTION('ref_axis',(1.,0.,0.));
#9571=DIRECTION('center_axis',(1.,0.,0.));
#9572=DIRECTION('ref_axis',(0.,-1.22464679914735E-16,1.));
#9573=DIRECTION('',(1.,0.,0.));
#9574=DIRECTION('center_axis',(1.,0.,0.));
#9575=DIRECTION('ref_axis',(0.,0.,-1.));
#9576=DIRECTION('',(-1.,0.,0.));
#9577=DIRECTION('center_axis',(1.,0.,0.));
#9578=DIRECTION('ref_axis',(0.,0.,-1.));
#9579=DIRECTION('center_axis',(1.,0.,0.));
#9580=DIRECTION('ref_axis',(0.,0.,-1.));
#9581=DIRECTION('',(0.,-1.,0.));
#9582=DIRECTION('center_axis',(-1.,0.,0.));
#9583=DIRECTION('ref_axis',(0.,-1.,0.));
#9584=DIRECTION('',(0.,-1.,0.));
#9585=DIRECTION('',(0.,0.,1.));
#9586=DIRECTION('',(0.,1.,0.));
#9587=DIRECTION('center_axis',(1.,0.,0.));
#9588=DIRECTION('ref_axis',(0.,0.,-1.));
#9589=DIRECTION('',(0.,1.,0.));
#9590=DIRECTION('',(0.,1.,0.));
#9591=DIRECTION('center_axis',(1.,0.,0.));
#9592=DIRECTION('ref_axis',(0.,0.,-1.));
#9593=DIRECTION('center_axis',(1.,0.,0.));
#9594=DIRECTION('ref_axis',(0.,0.,-1.));
#9595=DIRECTION('center_axis',(-1.,0.,0.));
#9596=DIRECTION('ref_axis',(0.,0.,-1.));
#9597=DIRECTION('center_axis',(1.,0.,0.));
#9598=DIRECTION('ref_axis',(0.,0.,-1.));
#9599=DIRECTION('center_axis',(1.,0.,0.));
#9600=DIRECTION('ref_axis',(0.,0.,-1.));
#9601=DIRECTION('',(1.,0.,0.));
#9602=DIRECTION('center_axis',(-1.,0.,0.));
#9603=DIRECTION('ref_axis',(0.,0.,-1.));
#9604=DIRECTION('center_axis',(0.,0.,1.));
#9605=DIRECTION('ref_axis',(1.,0.,0.));
#9606=DIRECTION('',(-1.,0.,0.));
#9607=DIRECTION('',(0.,-1.,0.));
#9608=DIRECTION('',(1.,0.,0.));
#9609=DIRECTION('',(0.,1.,0.));
#9610=DIRECTION('',(1.,0.,0.));
#9611=DIRECTION('',(0.,-1.,0.));
#9612=DIRECTION('',(-1.,0.,0.));
#9613=DIRECTION('',(0.,1.,0.));
#9614=DIRECTION('center_axis',(1.,0.,0.));
#9615=DIRECTION('ref_axis',(0.,0.,-1.));
#9616=DIRECTION('',(1.,0.,0.));
#9617=DIRECTION('center_axis',(-1.,0.,0.));
#9618=DIRECTION('ref_axis',(0.,0.,-1.));
#9619=DIRECTION('center_axis',(1.,0.,0.));
#9620=DIRECTION('ref_axis',(0.,-1.22464679914735E-16,1.));
#9621=DIRECTION('center_axis',(1.,0.,0.));
#9622=DIRECTION('ref_axis',(0.,0.,-1.));
#9623=DIRECTION('center_axis',(1.,0.,0.));
#9624=DIRECTION('ref_axis',(0.,0.,-1.));
#9625=DIRECTION('center_axis',(1.,0.,0.));
#9626=DIRECTION('ref_axis',(0.,0.,-1.));
#9627=DIRECTION('',(1.,0.,0.));
#9628=DIRECTION('center_axis',(-1.,0.,0.));
#9629=DIRECTION('ref_axis',(0.,0.,-1.));
#9630=DIRECTION('center_axis',(1.,0.,0.));
#9631=DIRECTION('ref_axis',(0.,0.,-1.));
#9632=DIRECTION('',(1.,0.,0.));
#9633=DIRECTION('center_axis',(-1.,0.,0.));
#9634=DIRECTION('ref_axis',(0.,0.,-1.));
#9635=DIRECTION('center_axis',(1.,0.,0.));
#9636=DIRECTION('ref_axis',(0.,1.,0.));
#9637=DIRECTION('',(0.,0.,1.));
#9638=DIRECTION('',(0.,1.,0.));
#9639=DIRECTION('',(0.,0.,1.));
#9640=DIRECTION('center_axis',(1.,0.,0.));
#9641=DIRECTION('ref_axis',(0.,1.,0.));
#9642=DIRECTION('',(0.,0.,1.));
#9643=DIRECTION('',(0.,1.,0.));
#9644=DIRECTION('center_axis',(0.,1.,0.));
#9645=DIRECTION('ref_axis',(-1.,0.,0.));
#9646=DIRECTION('',(0.,0.,1.));
#9647=DIRECTION('',(-1.,0.,0.));
#9648=DIRECTION('center_axis',(0.,-1.,0.));
#9649=DIRECTION('ref_axis',(1.,0.,0.));
#9650=DIRECTION('',(1.,0.,0.));
#9651=DIRECTION('',(0.,0.,1.));
#9652=DIRECTION('center_axis',(-1.,0.,0.));
#9653=DIRECTION('ref_axis',(0.,-1.,0.));
#9654=DIRECTION('',(0.,-1.,0.));
#9655=DIRECTION('center_axis',(0.,0.,1.));
#9656=DIRECTION('ref_axis',(1.,0.,0.));
#9657=DIRECTION('',(0.,-1.,0.));
#9658=DIRECTION('center_axis',(-1.,0.,0.));
#9659=DIRECTION('ref_axis',(0.,-1.,0.));
#9660=DIRECTION('',(0.,0.,1.));
#9661=DIRECTION('',(0.,-1.,0.));
#9662=DIRECTION('center_axis',(1.,0.,0.));
#9663=DIRECTION('ref_axis',(0.,1.,0.));
#9664=DIRECTION('',(0.,1.,0.));
#9665=DIRECTION('',(0.,0.,1.));
#9666=DIRECTION('',(0.,1.,0.));
#9667=DIRECTION('center_axis',(0.,-1.,0.));
#9668=DIRECTION('ref_axis',(1.,0.,0.));
#9669=DIRECTION('',(1.,0.,0.));
#9670=DIRECTION('',(1.,0.,0.));
#9671=DIRECTION('center_axis',(0.,0.,1.));
#9672=DIRECTION('ref_axis',(1.,0.,0.));
#9673=DIRECTION('center_axis',(0.,0.,1.));
#9674=DIRECTION('ref_axis',(1.,0.,0.));
#14214=CARTESIAN_POINT('',(0.,0.,0.));
#14215=CARTESIAN_POINT('Origin',(-2.1,3.,17.6));
#14216=CARTESIAN_POINT('',(-2.,3.,17.825));
#14217=CARTESIAN_POINT('Origin',(-2.,3.,17.6));
#14218=CARTESIAN_POINT('',(-1.2,3.,17.825));
#14219=CARTESIAN_POINT('',(-2.1,3.,17.825));
#14220=CARTESIAN_POINT('Origin',(-1.2,3.,17.6));
#14221=CARTESIAN_POINT('Origin',(-1.6,3.,17.));
#14222=CARTESIAN_POINT('',(-2.,3.,17.));
#14223=CARTESIAN_POINT('',(-1.2,3.,17.));
#14224=CARTESIAN_POINT('',(-1.4,3.,17.));
#14225=CARTESIAN_POINT('',(-2.,3.6,17.));
#14226=CARTESIAN_POINT('',(-2.,3.6,17.));
#14227=CARTESIAN_POINT('',(-1.2,3.6,17.));
#14228=CARTESIAN_POINT('',(-1.2,3.6,17.));
#14229=CARTESIAN_POINT('',(-1.2,2.4,17.));
#14230=CARTESIAN_POINT('Origin',(-1.2,3.6,17.));
#14231=CARTESIAN_POINT('',(-2.,3.6,18.2));
#14232=CARTESIAN_POINT('',(-2.,3.6,17.));
#14233=CARTESIAN_POINT('',(-1.2,3.6,18.2));
#14234=CARTESIAN_POINT('',(-1.2,3.6,18.2));
#14235=CARTESIAN_POINT('',(-1.2,3.6,17.));
#14236=CARTESIAN_POINT('Origin',(-1.6,3.,18.2));
#14237=CARTESIAN_POINT('',(-1.2,3.,18.2));
#14238=CARTESIAN_POINT('',(-2.,3.,18.2));
#14239=CARTESIAN_POINT('',(-1.4,3.,18.2));
#14240=CARTESIAN_POINT('',(-1.2,2.4,18.2));
#14241=CARTESIAN_POINT('',(-2.,3.6,18.2));
#14242=CARTESIAN_POINT('Origin',(-1.2,3.,16.));
#14243=CARTESIAN_POINT('',(-1.2,3.,16.));
#14244=CARTESIAN_POINT('',(-1.2,3.,16.));
#14245=CARTESIAN_POINT('',(-2.,3.,16.));
#14246=CARTESIAN_POINT('',(-1.2,3.,16.));
#14247=CARTESIAN_POINT('',(-2.,3.,16.));
#14248=CARTESIAN_POINT('Origin',(-1.2,3.,16.));
#14249=CARTESIAN_POINT('',(-2.,3.,21.));
#14250=CARTESIAN_POINT('',(-2.,3.,16.));
#14251=CARTESIAN_POINT('',(-2.,3.,22.));
#14252=CARTESIAN_POINT('',(-2.,3.,16.));
#14253=CARTESIAN_POINT('',(-2.,3.,23.));
#14254=CARTESIAN_POINT('',(-2.,3.,16.));
#14255=CARTESIAN_POINT('',(-1.2,3.,23.));
#14256=CARTESIAN_POINT('',(-1.2,3.,23.));
#14257=CARTESIAN_POINT('',(-1.2,3.,16.));
#14258=CARTESIAN_POINT('Origin',(-7.,0.,20.9));
#14259=CARTESIAN_POINT('',(-7.525,-6.42939569552361E-17,21.));
#14260=CARTESIAN_POINT('Origin',(-7.,0.,21.));
#14261=CARTESIAN_POINT('',(-7.525,6.42939569552361E-17,22.));
#14262=CARTESIAN_POINT('',(-7.525,-6.42939569552361E-17,20.9));
#14263=CARTESIAN_POINT('Origin',(-7.,0.,22.));
#14264=CARTESIAN_POINT('Origin',(-5.2,0.,20.9));
#14265=CARTESIAN_POINT('',(-5.65,-5.51091059616309E-17,21.));
#14266=CARTESIAN_POINT('Origin',(-5.2,0.,21.));
#14267=CARTESIAN_POINT('',(-5.65,5.51091059616309E-17,22.));
#14268=CARTESIAN_POINT('',(-5.65,-5.51091059616309E-17,20.9));
#14269=CARTESIAN_POINT('Origin',(-5.2,0.,22.));
#14270=CARTESIAN_POINT('Origin',(-8.8,0.,20.9));
#14271=CARTESIAN_POINT('',(-9.25,-5.51091059616308E-17,21.));
#14272=CARTESIAN_POINT('Origin',(-8.8,0.,21.));
#14273=CARTESIAN_POINT('',(-9.25,5.51091059616308E-17,22.));
#14274=CARTESIAN_POINT('',(-9.25,-5.51091059616308E-17,20.9));
#14275=CARTESIAN_POINT('Origin',(-8.8,0.,22.));
#14276=CARTESIAN_POINT('Origin',(-2.7,1.9,21.));
#14277=CARTESIAN_POINT('',(-2.7,1.4,21.));
#14278=CARTESIAN_POINT('',(-2.,1.4,21.));
#14279=CARTESIAN_POINT('',(-2.7,1.4,21.));
#14280=CARTESIAN_POINT('',(-2.7,2.4,21.));
#14281=CARTESIAN_POINT('Origin',(-2.7,1.9,21.));
#14282=CARTESIAN_POINT('',(-2.,2.4,21.));
#14283=CARTESIAN_POINT('',(-2.7,2.4,21.));
#14284=CARTESIAN_POINT('Origin',(-2.,1.9,21.));
#14285=CARTESIAN_POINT('Origin',(-2.7,1.9,21.));
#14286=CARTESIAN_POINT('',(-2.7,0.95,21.));
#14287=CARTESIAN_POINT('Origin',(-2.,3.,16.));
#14288=CARTESIAN_POINT('',(-2.,-3.,16.));
#14289=CARTESIAN_POINT('',(-2.,3.,16.));
#14290=CARTESIAN_POINT('',(-2.,-3.,21.));
#14291=CARTESIAN_POINT('',(-2.,-3.,16.));
#14292=CARTESIAN_POINT('',(-2.,-2.4,21.));
#14293=CARTESIAN_POINT('',(-2.,1.5,21.));
#14294=CARTESIAN_POINT('',(-2.,-1.4,21.));
#14295=CARTESIAN_POINT('Origin',(-2.,-1.9,21.));
#14296=CARTESIAN_POINT('',(-2.,1.5,21.));
#14297=CARTESIAN_POINT('',(-2.,1.5,21.));
#14298=CARTESIAN_POINT('',(-2.,1.9,21.275));
#14299=CARTESIAN_POINT('Origin',(-2.,1.9,21.));
#14300=CARTESIAN_POINT('',(-2.,-1.9,18.275));
#14301=CARTESIAN_POINT('Origin',(-2.,-1.9,18.));
#14302=CARTESIAN_POINT('',(-2.,-1.9,21.275));
#14303=CARTESIAN_POINT('Origin',(-2.,-1.9,21.));
#14304=CARTESIAN_POINT('',(-2.,1.9,18.275));
#14305=CARTESIAN_POINT('Origin',(-2.,1.9,18.));
#14306=CARTESIAN_POINT('Origin',(-2.1,1.9,21.));
#14307=CARTESIAN_POINT('',(-1.2,1.9,21.275));
#14308=CARTESIAN_POINT('',(-2.1,1.9,21.275));
#14309=CARTESIAN_POINT('Origin',(-1.2,1.9,21.));
#14310=CARTESIAN_POINT('Origin',(-7.,0.,21.));
#14311=CARTESIAN_POINT('',(-2.7,-1.4,21.));
#14312=CARTESIAN_POINT('',(-2.7,-1.4,21.));
#14313=CARTESIAN_POINT('',(-2.7,-2.4,21.));
#14314=CARTESIAN_POINT('',(-2.7,-0.95,21.));
#14315=CARTESIAN_POINT('',(-2.7,-2.4,21.));
#14316=CARTESIAN_POINT('',(-2.,-6.,21.));
#14317=CARTESIAN_POINT('',(-2.,-6.,21.));
#14318=CARTESIAN_POINT('',(-12.,-6.,21.));
#14319=CARTESIAN_POINT('',(-12.,-6.,21.));
#14320=CARTESIAN_POINT('',(-12.,6.,21.));
#14321=CARTESIAN_POINT('',(-12.,6.,21.));
#14322=CARTESIAN_POINT('',(-2.,6.,21.));
#14323=CARTESIAN_POINT('',(-2.,6.,21.));
#14324=CARTESIAN_POINT('',(-2.,-6.,21.));
#14325=CARTESIAN_POINT('Origin',(-2.1,1.9,18.));
#14326=CARTESIAN_POINT('',(-1.2,1.9,18.275));
#14327=CARTESIAN_POINT('',(-2.1,1.9,18.275));
#14328=CARTESIAN_POINT('Origin',(-1.2,1.9,18.));
#14329=CARTESIAN_POINT('Origin',(-2.7,-1.9,21.));
#14330=CARTESIAN_POINT('Origin',(-2.7,-1.9,21.));
#14331=CARTESIAN_POINT('Origin',(-2.7,-1.9,21.));
#14332=CARTESIAN_POINT('Origin',(-2.1,-1.9,21.));
#14333=CARTESIAN_POINT('',(-1.2,-1.9,21.275));
#14334=CARTESIAN_POINT('',(-2.1,-1.9,21.275));
#14335=CARTESIAN_POINT('Origin',(-1.2,-1.9,21.));
#14336=CARTESIAN_POINT('Origin',(-2.1,-1.9,18.));
#14337=CARTESIAN_POINT('',(-1.2,-1.9,18.275));
#14338=CARTESIAN_POINT('',(-2.1,-1.9,18.275));
#14339=CARTESIAN_POINT('Origin',(-1.2,-1.9,18.));
#14340=CARTESIAN_POINT('Origin',(-2.,-6.,21.));
#14341=CARTESIAN_POINT('',(-2.,-3.,22.));
#14342=CARTESIAN_POINT('',(-2.,-3.,16.));
#14343=CARTESIAN_POINT('',(-2.,-6.,22.));
#14344=CARTESIAN_POINT('',(-2.,-6.,22.));
#14345=CARTESIAN_POINT('',(-2.,-6.,21.));
#14346=CARTESIAN_POINT('Origin',(-2.,-6.,21.));
#14347=CARTESIAN_POINT('',(-2.,6.,22.));
#14348=CARTESIAN_POINT('',(-2.,6.,21.));
#14349=CARTESIAN_POINT('',(-2.,-6.,22.));
#14350=CARTESIAN_POINT('Origin',(-2.,6.,21.));
#14351=CARTESIAN_POINT('',(-12.,6.,22.));
#14352=CARTESIAN_POINT('',(-12.,6.,21.));
#14353=CARTESIAN_POINT('',(-2.,6.,22.));
#14354=CARTESIAN_POINT('Origin',(-12.,-6.,21.));
#14355=CARTESIAN_POINT('',(-12.,-6.,22.));
#14356=CARTESIAN_POINT('',(-12.,-6.,22.));
#14357=CARTESIAN_POINT('',(-12.,-6.,21.));
#14358=CARTESIAN_POINT('Origin',(-12.,6.,21.));
#14359=CARTESIAN_POINT('',(-12.,6.,22.));
#14360=CARTESIAN_POINT('Origin',(-7.,0.,22.));
#14361=CARTESIAN_POINT('',(-2.,1.5,22.));
#14362=CARTESIAN_POINT('Origin',(-2.,3.,16.));
#14363=CARTESIAN_POINT('',(-2.,-3.,23.));
#14364=CARTESIAN_POINT('',(-2.,-3.,16.));
#14365=CARTESIAN_POINT('',(-2.,3.,23.));
#14366=CARTESIAN_POINT('Origin',(-1.2,-3.,16.));
#14367=CARTESIAN_POINT('',(-1.2,-3.,23.));
#14368=CARTESIAN_POINT('',(-1.2,-3.,23.));
#14369=CARTESIAN_POINT('',(-1.2,-3.,16.));
#14370=CARTESIAN_POINT('',(-1.2,-3.,16.));
#14371=CARTESIAN_POINT('',(-1.2,-3.,16.));
#14372=CARTESIAN_POINT('Origin',(-2.,-3.,16.));
#14373=CARTESIAN_POINT('',(-2.,-3.,16.));
#14374=CARTESIAN_POINT('',(-2.,-3.,23.));
#14375=CARTESIAN_POINT('Origin',(-1.6,0.,23.));
#14376=CARTESIAN_POINT('Origin',(-1.6,0.,16.));
#14987=UNCERTAINTY_MEASURE_WITH_UNIT(LENGTH_MEASURE(0.001),#15041,
'DISTANCE_ACCURACY_VALUE',
'Maximum model space distance between geometric entities at asserted c
onnectivities');
#15000=UNCERTAINTY_MEASURE_WITH_UNIT(LENGTH_MEASURE(0.001),#15041,
'DISTANCE_ACCURACY_VALUE',
'Maximum model space distance between geometric entities at asserted c
onnectivities');
#15027=(
GEOMETRIC_REPRESENTATION_CONTEXT(3)
GLOBAL_UNCERTAINTY_ASSIGNED_CONTEXT((#14987))
GLOBAL_UNIT_ASSIGNED_CONTEXT((#15041,#15043,#15044))
REPRESENTATION_CONTEXT('','3D')
);
#15040=(
GEOMETRIC_REPRESENTATION_CONTEXT(3)
GLOBAL_UNCERTAINTY_ASSIGNED_CONTEXT((#15000))
GLOBAL_UNIT_ASSIGNED_CONTEXT((#15041,#15043,#15044))
REPRESENTATION_CONTEXT('','3D')
);
#15041=(
LENGTH_UNIT()
NAMED_UNIT(*)
SI_UNIT(.CENTI.,.METRE.)
);
#15043=(
NAMED_UNIT(*)
PLANE_ANGLE_UNIT()
SI_UNIT($,.RADIAN.)
);
#15044=(
NAMED_UNIT(*)
SI_UNIT($,.STERADIAN.)
SOLID_ANGLE_UNIT()
);
#15071=SHAPE_DEFINITION_REPRESENTATION(#15110,#15208);
#15110=PRODUCT_DEFINITION_SHAPE('',$,#15248);
#15208=SHAPE_REPRESENTATION('',(#7932),#15027);
#15221=PRODUCT_DEFINITION_CONTEXT('part definition',#15340,'design');
#15248=PRODUCT_DEFINITION('Platform and carriage bracket',
'Platform and carriage bracket',#15287,#15221);
#15287=PRODUCT_DEFINITION_FORMATION('',$,#15368);
#15340=APPLICATION_CONTEXT(
'Core Data for Automotive Mechanical Design Process');
#15341=PRODUCT_CONTEXT('part definition',#15340,'mechanical');
#15368=PRODUCT('Platform and carriage bracket',
'Platform and carriage bracket','Platform and carriage bracket',(#15341));
#15430=COLOUR_RGB('Dark Blue',0.08,0.2,0.34);
#15431=FILL_AREA_STYLE_COLOUR('',#15430);
#15432=FILL_AREA_STYLE('',(#15431));
#15433=SURFACE_STYLE_FILL_AREA(#15432);
#15434=SURFACE_SIDE_STYLE('',(#15433));
#15435=SURFACE_STYLE_USAGE(.BOTH.,#15434);
#15436=PRESENTATION_STYLE_ASSIGNMENT((#15435));
ENDSEC;
END-ISO-10303-21;
